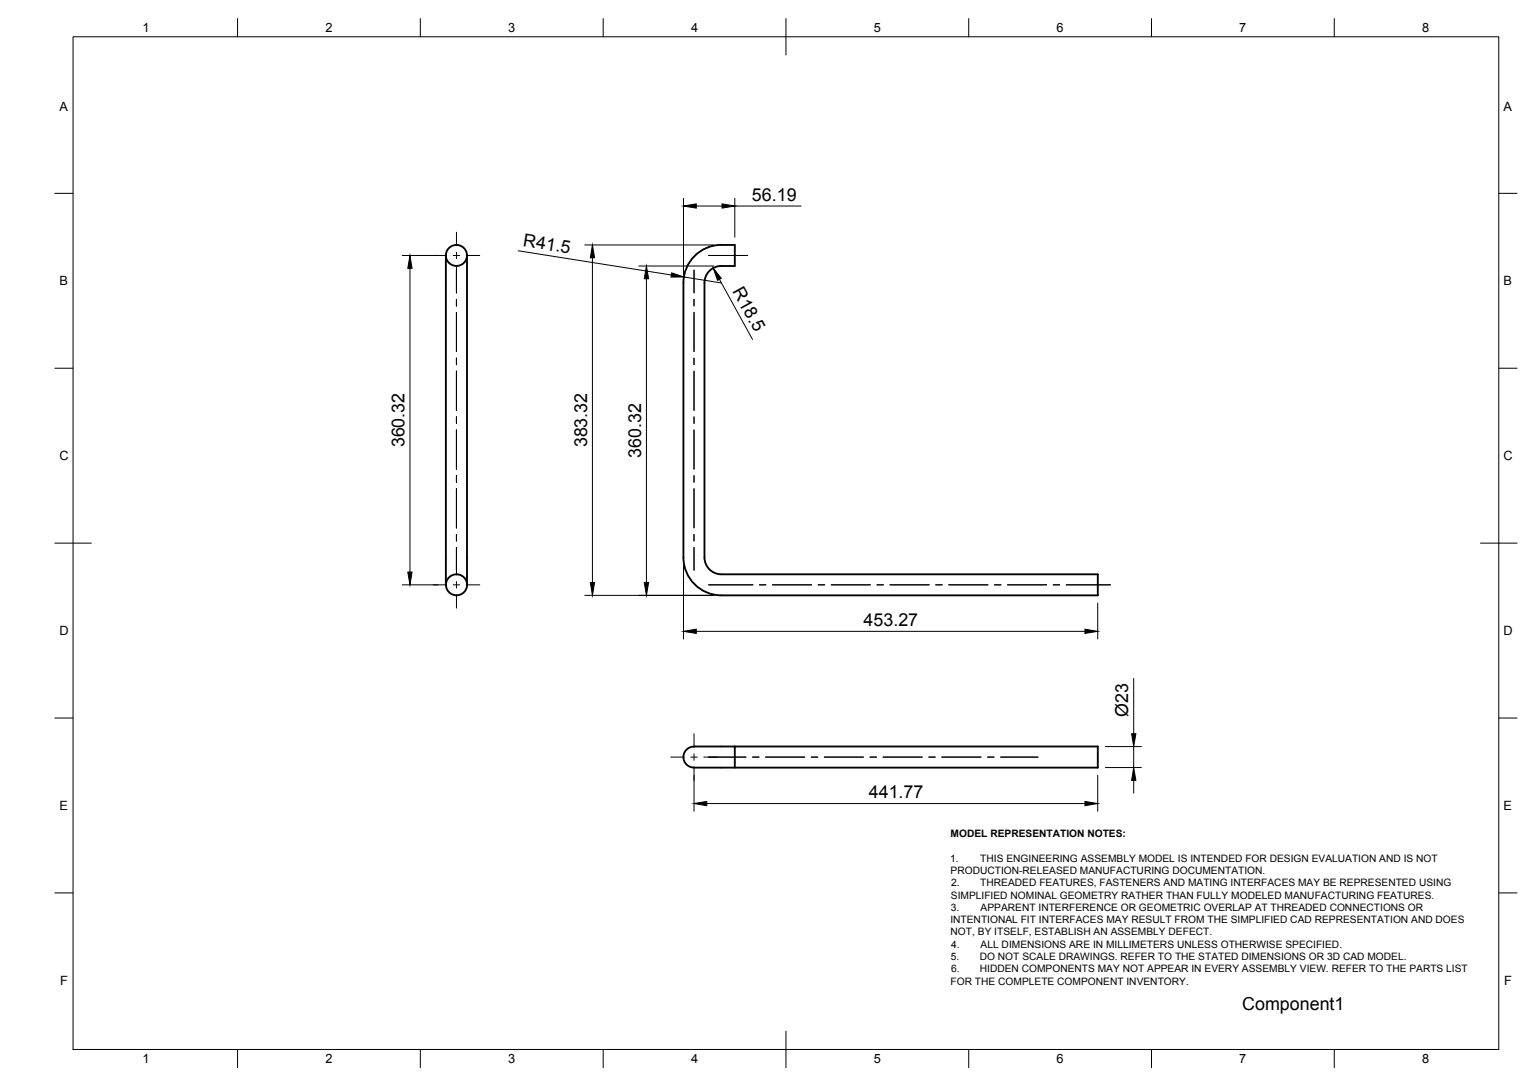
ISO-10303-21;
HEADER;
/* Generated by software containing ST-Developer
 * from STEP Tools, Inc. (www.steptools.com) 
 */

FILE_DESCRIPTION(
/* description */ ('STEP AP214'),
/* implementation_level */ '2;1');

FILE_NAME(
/* name */ 'Component1.step',
/* time_stamp */ '2026-10-06T11:02:40-07:00',
/* author */ (''),
/* organization */ (''),
/* preprocessor_version */ 'ST-DEVELOPER v20.2',
/* originating_system */ 'Autodesk Translation Framework v15.15.0.0',
/* authorisation */ '');

FILE_SCHEMA (('AUTOMOTIVE_DESIGN { 1 0 10303 214 3 1 1 }'));
ENDSEC;

DATA;
#10=MECHANICAL_DESIGN_GEOMETRIC_PRESENTATION_REPRESENTATION('',(#2936),#130910);
#2920=SHAPE_REPRESENTATION_RELATIONSHIP('SRR','None',#130942,#2928);
#2928=ADVANCED_BREP_SHAPE_REPRESENTATION('',(#2944),#130902);
#2936=STYLED_ITEM('',(#130991),#2944);
#2944=MANIFOLD_SOLID_BREP('Body1',#45448);
#2950=PLANE('',#45566);
#2951=PLANE('',#45567);
#4312=LINE('',#65500,#6086);
#4313=LINE('',#65502,#6087);
#4314=LINE('',#65505,#6088);
#6086=VECTOR('',#51629,11.5);
#6087=VECTOR('',#51632,11.5);
#6088=VECTOR('',#51635,11.5);
#7860=CYLINDRICAL_SURFACE('',#45561,11.5);
#7861=CYLINDRICAL_SURFACE('',#45563,11.5);
#7862=CYLINDRICAL_SURFACE('',#45564,11.5);
#9467=FACE_OUTER_BOUND('',#12868,.T.);
#9468=FACE_OUTER_BOUND('',#12869,.T.);
#9469=FACE_OUTER_BOUND('',#12870,.T.);
#9470=FACE_OUTER_BOUND('',#12871,.T.);
#9471=FACE_OUTER_BOUND('',#12872,.T.);
#9472=FACE_OUTER_BOUND('',#12873,.T.);
#9473=FACE_OUTER_BOUND('',#12874,.T.);
#12868=EDGE_LOOP('',(#30316,#30317,#30318,#30319,#30320));
#12869=EDGE_LOOP('',(#30321,#30322,#30323,#30324,#30325));
#12870=EDGE_LOOP('',(#30326,#30327,#30328,#30329));
#12871=EDGE_LOOP('',(#30330,#30331,#30332,#30333,#30334,#30335));
#12872=EDGE_LOOP('',(#30336,#30337,#30338,#30339));
#12873=EDGE_LOOP('',(#30340));
#12874=EDGE_LOOP('',(#30341));
#17703=CIRCLE('',#45552,11.5);
#17704=CIRCLE('',#45553,18.5);
#17705=CIRCLE('',#45554,11.5000000000001);
#17706=CIRCLE('',#45555,11.5000000000001);
#17707=CIRCLE('',#45557,11.5000000000001);
#17708=CIRCLE('',#45558,18.4999999999957);
#17709=CIRCLE('',#45559,11.5);
#17710=CIRCLE('',#45560,11.5000000000001);
#17711=CIRCLE('',#45562,11.5);
#17712=CIRCLE('',#45565,11.5);
#20635=VERTEX_POINT('',#65482);
#20636=VERTEX_POINT('',#65484);
#20637=VERTEX_POINT('',#65486);
#20638=VERTEX_POINT('',#65490);
#20639=VERTEX_POINT('',#65491);
#20640=VERTEX_POINT('',#65493);
#20641=VERTEX_POINT('',#65498);
#20642=VERTEX_POINT('',#65504);
#24502=EDGE_CURVE('',#20635,#20635,#17703,.T.);
#24503=EDGE_CURVE('',#20635,#20636,#17704,.T.);
#24504=EDGE_CURVE('',#20636,#20637,#17705,.T.);
#24505=EDGE_CURVE('',#20637,#20636,#17706,.T.);
#24506=EDGE_CURVE('',#20638,#20639,#17707,.T.);
#24507=EDGE_CURVE('',#20638,#20640,#17708,.T.);
#24508=EDGE_CURVE('',#20640,#20640,#17709,.T.);
#24509=EDGE_CURVE('',#20639,#20638,#17710,.T.);
#24510=EDGE_CURVE('',#20641,#20641,#17711,.T.);
#24511=EDGE_CURVE('',#20641,#20635,#4312,.T.);
#24512=EDGE_CURVE('',#20637,#20639,#4313,.T.);
#24513=EDGE_CURVE('',#20640,#20642,#4314,.T.);
#24514=EDGE_CURVE('',#20642,#20642,#17712,.T.);
#30316=ORIENTED_EDGE('',*,*,#24502,.F.);
#30317=ORIENTED_EDGE('',*,*,#24503,.T.);
#30318=ORIENTED_EDGE('',*,*,#24504,.T.);
#30319=ORIENTED_EDGE('',*,*,#24505,.T.);
#30320=ORIENTED_EDGE('',*,*,#24503,.F.);
#30321=ORIENTED_EDGE('',*,*,#24506,.F.);
#30322=ORIENTED_EDGE('',*,*,#24507,.T.);
#30323=ORIENTED_EDGE('',*,*,#24508,.T.);
#30324=ORIENTED_EDGE('',*,*,#24507,.F.);
#30325=ORIENTED_EDGE('',*,*,#24509,.F.);
#30326=ORIENTED_EDGE('',*,*,#24510,.T.);
#30327=ORIENTED_EDGE('',*,*,#24511,.T.);
#30328=ORIENTED_EDGE('',*,*,#24502,.T.);
#30329=ORIENTED_EDGE('',*,*,#24511,.F.);
#30330=ORIENTED_EDGE('',*,*,#24504,.F.);
#30331=ORIENTED_EDGE('',*,*,#24505,.F.);
#30332=ORIENTED_EDGE('',*,*,#24512,.T.);
#30333=ORIENTED_EDGE('',*,*,#24509,.T.);
#30334=ORIENTED_EDGE('',*,*,#24506,.T.);
#30335=ORIENTED_EDGE('',*,*,#24512,.F.);
#30336=ORIENTED_EDGE('',*,*,#24508,.F.);
#30337=ORIENTED_EDGE('',*,*,#24513,.T.);
#30338=ORIENTED_EDGE('',*,*,#24514,.T.);
#30339=ORIENTED_EDGE('',*,*,#24513,.F.);
#30340=ORIENTED_EDGE('',*,*,#24510,.F.);
#30341=ORIENTED_EDGE('',*,*,#24514,.F.);
#41944=TOROIDAL_SURFACE('',#45551,30.,11.5);
#41945=TOROIDAL_SURFACE('',#45556,29.9999999999957,11.5);
#42047=ADVANCED_FACE('',(#9467),#41944,.T.);
#42048=ADVANCED_FACE('',(#9468),#41945,.T.);
#42049=ADVANCED_FACE('',(#9469),#7860,.T.);
#42050=ADVANCED_FACE('',(#9470),#7861,.T.);
#42051=ADVANCED_FACE('',(#9471),#7862,.T.);
#42052=ADVANCED_FACE('',(#9472),#2950,.F.);
#42053=ADVANCED_FACE('',(#9473),#2951,.F.);
#45448=CLOSED_SHELL('',(#42047,#42048,#42049,#42050,#42051,#42052,#42053));
#45550=AXIS2_PLACEMENT_3D('',#65480,#51603,#51604);
#45551=AXIS2_PLACEMENT_3D('',#65481,#51605,#51606);
#45552=AXIS2_PLACEMENT_3D('',#65483,#51607,#51608);
#45553=AXIS2_PLACEMENT_3D('',#65485,#51609,#51610);
#45554=AXIS2_PLACEMENT_3D('',#65487,#51611,#51612);
#45555=AXIS2_PLACEMENT_3D('',#65488,#51613,#51614);
#45556=AXIS2_PLACEMENT_3D('',#65489,#51615,#51616);
#45557=AXIS2_PLACEMENT_3D('',#65492,#51617,#51618);
#45558=AXIS2_PLACEMENT_3D('',#65494,#51619,#51620);
#45559=AXIS2_PLACEMENT_3D('',#65495,#51621,#51622);
#45560=AXIS2_PLACEMENT_3D('',#65496,#51623,#51624);
#45561=AXIS2_PLACEMENT_3D('',#65497,#51625,#51626);
#45562=AXIS2_PLACEMENT_3D('',#65499,#51627,#51628);
#45563=AXIS2_PLACEMENT_3D('',#65501,#51630,#51631);
#45564=AXIS2_PLACEMENT_3D('',#65503,#51633,#51634);
#45565=AXIS2_PLACEMENT_3D('',#65506,#51636,#51637);
#45566=AXIS2_PLACEMENT_3D('',#65507,#51638,#51639);
#45567=AXIS2_PLACEMENT_3D('',#65508,#51640,#51641);
#51603=DIRECTION('axis',(0.,0.,1.));
#51604=DIRECTION('refdir',(1.,0.,0.));
#51605=DIRECTION('center_axis',(-1.,0.,0.));
#51606=DIRECTION('ref_axis',(0.,0.,1.));
#51607=DIRECTION('center_axis',(0.,-1.,-3.7789907496129E-15));
#51608=DIRECTION('ref_axis',(0.,3.7789907496129E-15,-1.));
#51609=DIRECTION('center_axis',(1.,0.,0.));
#51610=DIRECTION('ref_axis',(0.,0.,1.));
#51611=DIRECTION('center_axis',(0.,3.7789907496129E-15,-1.));
#51612=DIRECTION('ref_axis',(0.,1.,3.7789907496129E-15));
#51613=DIRECTION('center_axis',(0.,3.7789907496129E-15,-1.));
#51614=DIRECTION('ref_axis',(0.,1.,3.7789907496129E-15));
#51615=DIRECTION('center_axis',(-1.,0.,0.));
#51616=DIRECTION('ref_axis',(0.,0.,1.));
#51617=DIRECTION('center_axis',(0.,3.7789907496129E-15,-1.));
#51618=DIRECTION('ref_axis',(0.,1.,3.7789907496129E-15));
#51619=DIRECTION('center_axis',(1.,0.,0.));
#51620=DIRECTION('ref_axis',(0.,0.,1.));
#51621=DIRECTION('center_axis',(0.,1.,0.));
#51622=DIRECTION('ref_axis',(0.,0.,1.));
#51623=DIRECTION('center_axis',(0.,3.7789907496129E-15,-1.));
#51624=DIRECTION('ref_axis',(0.,1.,3.7789907496129E-15));
#51625=DIRECTION('center_axis',(0.,-1.,0.));
#51626=DIRECTION('ref_axis',(0.,0.,-1.));
#51627=DIRECTION('center_axis',(0.,1.,0.));
#51628=DIRECTION('ref_axis',(0.,0.,1.));
#51629=DIRECTION('',(0.,1.,0.));
#51630=DIRECTION('center_axis',(0.,0.,-1.));
#51631=DIRECTION('ref_axis',(-1.,0.,0.));
#51632=DIRECTION('',(0.,0.,1.));
#51633=DIRECTION('center_axis',(0.,1.,-3.7789907496129E-15));
#51634=DIRECTION('ref_axis',(0.,3.7789907496129E-15,1.));
#51635=DIRECTION('',(0.,-1.,3.7789907496129E-15));
#51636=DIRECTION('center_axis',(0.,1.,0.));
#51637=DIRECTION('ref_axis',(0.,0.,1.));
#51638=DIRECTION('center_axis',(0.,1.,0.));
#51639=DIRECTION('ref_axis',(0.,0.,1.));
#51640=DIRECTION('center_axis',(0.,1.,0.));
#51641=DIRECTION('ref_axis',(0.,0.,1.));
#65480=CARTESIAN_POINT('',(0.,0.,0.));
#65481=CARTESIAN_POINT('Origin',(0.,1148.83458861821,94.2994740882088));
#65482=CARTESIAN_POINT('',(1.40834381901946E-15,1148.83458861821,75.7994740882088));
#65483=CARTESIAN_POINT('Origin',(0.,1148.83458861821,64.2994740882088));
#65484=CARTESIAN_POINT('',(1.40834381901946E-15,1167.33458861821,94.2994740882088));
#65485=CARTESIAN_POINT('Origin',(1.40834381901946E-15,1148.83458861821,
94.2994740882088));
#65486=CARTESIAN_POINT('',(11.5,1178.83458861821,94.2994740882088));
#65487=CARTESIAN_POINT('Origin',(0.,1178.83458861821,94.2994740882088));
#65488=CARTESIAN_POINT('Origin',(0.,1178.83458861821,94.2994740882088));
#65489=CARTESIAN_POINT('Origin',(0.,1148.83458861821,394.620242579854));
#65490=CARTESIAN_POINT('',(1.40834381901946E-15,1167.33458861821,394.620242579854));
#65491=CARTESIAN_POINT('',(11.5,1178.83458861821,394.620242579854));
#65492=CARTESIAN_POINT('Origin',(0.,1178.83458861821,394.620242579854));
#65493=CARTESIAN_POINT('',(1.40834381901946E-15,1148.83458861821,413.120242579854));
#65494=CARTESIAN_POINT('Origin',(1.40834381901946E-15,1148.83458861821,
394.620242579854));
#65495=CARTESIAN_POINT('Origin',(0.,1148.83458861821,424.620242579854));
#65496=CARTESIAN_POINT('Origin',(0.,1178.83458861821,394.620242579854));
#65497=CARTESIAN_POINT('Origin',(0.,1148.83458861821,64.2994740882088));
#65498=CARTESIAN_POINT('',(-1.40834381901946E-15,737.065928490981,75.7994740882088));
#65499=CARTESIAN_POINT('Origin',(0.,737.065928490981,64.2994740882088));
#65500=CARTESIAN_POINT('',(-1.40834381901946E-15,1148.83458861821,75.7994740882088));
#65501=CARTESIAN_POINT('Origin',(0.,1178.83458861821,394.620242579854));
#65502=CARTESIAN_POINT('',(11.5,1178.83458861821,394.620242579854));
#65503=CARTESIAN_POINT('Origin',(0.,1134.14517683891,424.620242579854));
#65504=CARTESIAN_POINT('',(-1.40834381901946E-15,1134.14517683891,413.120242579854));
#65505=CARTESIAN_POINT('',(-1.40834381901946E-15,1134.14517683891,413.120242579854));
#65506=CARTESIAN_POINT('Origin',(0.,1134.14517683891,424.620242579854));
#65507=CARTESIAN_POINT('Origin',(0.,737.065928490981,76.7994740882088));
#65508=CARTESIAN_POINT('Origin',(0.,1134.14517683891,424.620242579854));
#130892=UNCERTAINTY_MEASURE_WITH_UNIT(LENGTH_MEASURE(0.01),#130911,
'DISTANCE_ACCURACY_VALUE',
'Maximum model space distance between geometric entities at asserted c
onnectivities');
#130900=UNCERTAINTY_MEASURE_WITH_UNIT(LENGTH_MEASURE(0.01),#130911,
'DISTANCE_ACCURACY_VALUE',
'Maximum model space distance between geometric entities at asserted c
onnectivities');
#130902=(
GEOMETRIC_REPRESENTATION_CONTEXT(3)
GLOBAL_UNCERTAINTY_ASSIGNED_CONTEXT((#130892))
GLOBAL_UNIT_ASSIGNED_CONTEXT((#130911,#130913,#130914))
REPRESENTATION_CONTEXT('','3D')
);
#130910=(
GEOMETRIC_REPRESENTATION_CONTEXT(3)
GLOBAL_UNCERTAINTY_ASSIGNED_CONTEXT((#130900))
GLOBAL_UNIT_ASSIGNED_CONTEXT((#130911,#130913,#130914))
REPRESENTATION_CONTEXT('','3D')
);
#130911=(
LENGTH_UNIT()
NAMED_UNIT(*)
SI_UNIT(.MILLI.,.METRE.)
);
#130913=(
NAMED_UNIT(*)
PLANE_ANGLE_UNIT()
SI_UNIT($,.RADIAN.)
);
#130914=(
NAMED_UNIT(*)
SI_UNIT($,.STERADIAN.)
SOLID_ANGLE_UNIT()
);
#130916=SHAPE_DEFINITION_REPRESENTATION(#130925,#130942);
#130925=PRODUCT_DEFINITION_SHAPE('',$,#130952);
#130942=SHAPE_REPRESENTATION('',(#45550),#130902);
#130950=PRODUCT_DEFINITION_CONTEXT('part definition',#130979,'design');
#130952=PRODUCT_DEFINITION('Component1','Component1',#130961,#130950);
#130961=PRODUCT_DEFINITION_FORMATION('',$,#130982);
#130979=APPLICATION_CONTEXT(
'Core Data for Automotive Mechanical Design Process');
#130980=PRODUCT_CONTEXT('part definition',#130979,'mechanical');
#130982=PRODUCT('Component1','Component1',$,(#130980));
#130991=PRESENTATION_STYLE_ASSIGNMENT((#130993));
#130993=SURFACE_STYLE_USAGE(.BOTH.,#130995);
#130995=SURFACE_SIDE_STYLE('',(#130997));
#130997=SURFACE_STYLE_FILL_AREA(#130999);
#130999=FILL_AREA_STYLE('Opaque(202,209,238)',(#131001));
#131001=FILL_AREA_STYLE_COLOUR('Opaque(202,209,238)',#131003);
#131003=COLOUR_RGB('Opaque(202,209,238)', 0.40784314, 0.44705882, 0.49803922);
ENDSEC;
END-ISO-10303-21;
